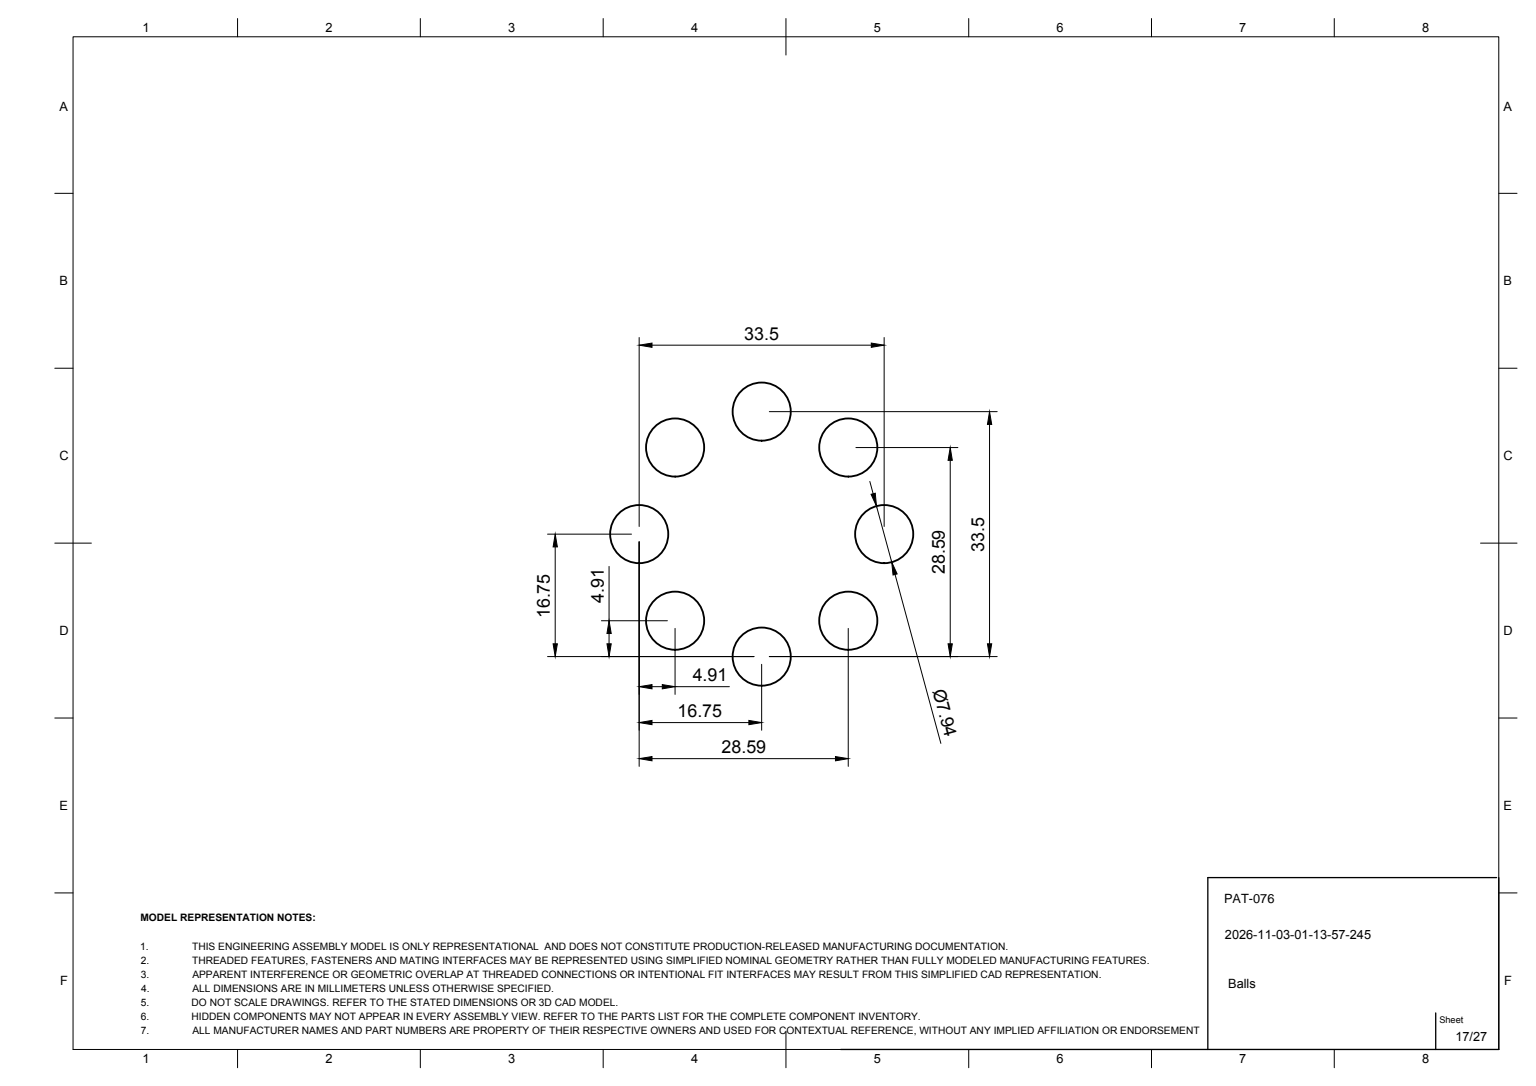
ISO-10303-21;
HEADER;
/* Generated by software containing ST-Developer
 * from STEP Tools, Inc. (www.steptools.com) 
 */

FILE_DESCRIPTION(
/* description */ ('Overhung pulley bearing cartridge'),
/* implementation_level */ '2;1');

FILE_NAME(
/* name */ 'Balls.step',
/* time_stamp */ '2026-10-28T03:22:33-07:00',
/* author */ (''),
/* organization */ (''),
/* preprocessor_version */ 'ST-DEVELOPER v20.2',
/* originating_system */ 'Autodesk Translation Framework v15.17.0.0',
/* authorisation */ '');

FILE_SCHEMA (('AUTOMOTIVE_DESIGN { 1 0 10303 214 3 1 1 }'));
ENDSEC;

DATA;
#10=MECHANICAL_DESIGN_GEOMETRIC_PRESENTATION_REPRESENTATION('',(#293,#294,#295,#296,#297,#298,#299,#300),#10963);
#207=SPHERICAL_SURFACE('',#6153,0.3969);
#208=SPHERICAL_SURFACE('',#6155,0.3969);
#209=SPHERICAL_SURFACE('',#6157,0.3969);
#210=SPHERICAL_SURFACE('',#6159,0.3969);
#211=SPHERICAL_SURFACE('',#6161,0.3969);
#212=SPHERICAL_SURFACE('',#6163,0.3969);
#213=SPHERICAL_SURFACE('',#6165,0.3969);
#214=SPHERICAL_SURFACE('',#6167,0.3969);
#249=SHAPE_REPRESENTATION_RELATIONSHIP('SRR','None',#11070,#271);
#271=ADVANCED_BREP_SHAPE_REPRESENTATION('',(#323,#324,#325,#326,#327,#328,
#329,#330),#10950);
#293=STYLED_ITEM('',(#11253),#323);
#294=STYLED_ITEM('',(#11253),#324);
#295=STYLED_ITEM('',(#11253),#325);
#296=STYLED_ITEM('',(#11253),#326);
#297=STYLED_ITEM('',(#11253),#327);
#298=STYLED_ITEM('',(#11253),#328);
#299=STYLED_ITEM('',(#11253),#329);
#300=STYLED_ITEM('',(#11253),#330);
#323=MANIFOLD_SOLID_BREP('Body1',#5660);
#324=MANIFOLD_SOLID_BREP('Body2',#5661);
#325=MANIFOLD_SOLID_BREP('Body3',#5662);
#326=MANIFOLD_SOLID_BREP('Body4',#5663);
#327=MANIFOLD_SOLID_BREP('Body5',#5664);
#328=MANIFOLD_SOLID_BREP('Body6',#5665);
#329=MANIFOLD_SOLID_BREP('Body7',#5666);
#330=MANIFOLD_SOLID_BREP('Body8',#5667);
#687=FACE_OUTER_BOUND('',#1075,.T.);
#688=FACE_OUTER_BOUND('',#1076,.T.);
#689=FACE_OUTER_BOUND('',#1077,.T.);
#690=FACE_OUTER_BOUND('',#1078,.T.);
#691=FACE_OUTER_BOUND('',#1079,.T.);
#692=FACE_OUTER_BOUND('',#1080,.T.);
#693=FACE_OUTER_BOUND('',#1081,.T.);
#694=FACE_OUTER_BOUND('',#1082,.T.);
#1075=EDGE_LOOP('',(#4099,#4100));
#1076=EDGE_LOOP('',(#4101,#4102));
#1077=EDGE_LOOP('',(#4103,#4104));
#1078=EDGE_LOOP('',(#4105,#4106));
#1079=EDGE_LOOP('',(#4107,#4108));
#1080=EDGE_LOOP('',(#4109,#4110));
#1081=EDGE_LOOP('',(#4111,#4112));
#1082=EDGE_LOOP('',(#4113,#4114));
#2116=CIRCLE('',#6154,0.3969);
#2117=CIRCLE('',#6156,0.3969);
#2118=CIRCLE('',#6158,0.3969);
#2119=CIRCLE('',#6160,0.3969);
#2120=CIRCLE('',#6162,0.3969);
#2121=CIRCLE('',#6164,0.3969);
#2122=CIRCLE('',#6166,0.3969);
#2123=CIRCLE('',#6168,0.3969);
#2529=VERTEX_POINT('',#9050);
#2530=VERTEX_POINT('',#9051);
#2531=VERTEX_POINT('',#9054);
#2532=VERTEX_POINT('',#9055);
#2533=VERTEX_POINT('',#9058);
#2534=VERTEX_POINT('',#9059);
#2535=VERTEX_POINT('',#9062);
#2536=VERTEX_POINT('',#9063);
#2537=VERTEX_POINT('',#9066);
#2538=VERTEX_POINT('',#9067);
#2539=VERTEX_POINT('',#9070);
#2540=VERTEX_POINT('',#9071);
#2541=VERTEX_POINT('',#9074);
#2542=VERTEX_POINT('',#9075);
#2543=VERTEX_POINT('',#9078);
#2544=VERTEX_POINT('',#9079);
#3119=EDGE_CURVE('',#2529,#2530,#2116,.T.);
#3120=EDGE_CURVE('',#2531,#2532,#2117,.T.);
#3121=EDGE_CURVE('',#2533,#2534,#2118,.T.);
#3122=EDGE_CURVE('',#2535,#2536,#2119,.T.);
#3123=EDGE_CURVE('',#2537,#2538,#2120,.T.);
#3124=EDGE_CURVE('',#2539,#2540,#2121,.T.);
#3125=EDGE_CURVE('',#2541,#2542,#2122,.T.);
#3126=EDGE_CURVE('',#2543,#2544,#2123,.T.);
#4099=ORIENTED_EDGE('',*,*,#3119,.T.);
#4100=ORIENTED_EDGE('',*,*,#3119,.F.);
#4101=ORIENTED_EDGE('',*,*,#3120,.T.);
#4102=ORIENTED_EDGE('',*,*,#3120,.F.);
#4103=ORIENTED_EDGE('',*,*,#3121,.T.);
#4104=ORIENTED_EDGE('',*,*,#3121,.F.);
#4105=ORIENTED_EDGE('',*,*,#3122,.T.);
#4106=ORIENTED_EDGE('',*,*,#3122,.F.);
#4107=ORIENTED_EDGE('',*,*,#3123,.T.);
#4108=ORIENTED_EDGE('',*,*,#3123,.F.);
#4109=ORIENTED_EDGE('',*,*,#3124,.T.);
#4110=ORIENTED_EDGE('',*,*,#3124,.F.);
#4111=ORIENTED_EDGE('',*,*,#3125,.T.);
#4112=ORIENTED_EDGE('',*,*,#3125,.F.);
#4113=ORIENTED_EDGE('',*,*,#3126,.T.);
#4114=ORIENTED_EDGE('',*,*,#3126,.F.);
#5431=ADVANCED_FACE('',(#687),#207,.T.);
#5432=ADVANCED_FACE('',(#688),#208,.T.);
#5433=ADVANCED_FACE('',(#689),#209,.T.);
#5434=ADVANCED_FACE('',(#690),#210,.T.);
#5435=ADVANCED_FACE('',(#691),#211,.T.);
#5436=ADVANCED_FACE('',(#692),#212,.T.);
#5437=ADVANCED_FACE('',(#693),#213,.T.);
#5438=ADVANCED_FACE('',(#694),#214,.T.);
#5660=CLOSED_SHELL('',(#5431));
#5661=CLOSED_SHELL('',(#5432));
#5662=CLOSED_SHELL('',(#5433));
#5663=CLOSED_SHELL('',(#5434));
#5664=CLOSED_SHELL('',(#5435));
#5665=CLOSED_SHELL('',(#5436));
#5666=CLOSED_SHELL('',(#5437));
#5667=CLOSED_SHELL('',(#5438));
#6152=AXIS2_PLACEMENT_3D('',#9048,#7261,#7262);
#6153=AXIS2_PLACEMENT_3D('',#9049,#7263,#7264);
#6154=AXIS2_PLACEMENT_3D('',#9052,#7265,#7266);
#6155=AXIS2_PLACEMENT_3D('',#9053,#7267,#7268);
#6156=AXIS2_PLACEMENT_3D('',#9056,#7269,#7270);
#6157=AXIS2_PLACEMENT_3D('',#9057,#7271,#7272);
#6158=AXIS2_PLACEMENT_3D('',#9060,#7273,#7274);
#6159=AXIS2_PLACEMENT_3D('',#9061,#7275,#7276);
#6160=AXIS2_PLACEMENT_3D('',#9064,#7277,#7278);
#6161=AXIS2_PLACEMENT_3D('',#9065,#7279,#7280);
#6162=AXIS2_PLACEMENT_3D('',#9068,#7281,#7282);
#6163=AXIS2_PLACEMENT_3D('',#9069,#7283,#7284);
#6164=AXIS2_PLACEMENT_3D('',#9072,#7285,#7286);
#6165=AXIS2_PLACEMENT_3D('',#9073,#7287,#7288);
#6166=AXIS2_PLACEMENT_3D('',#9076,#7289,#7290);
#6167=AXIS2_PLACEMENT_3D('',#9077,#7291,#7292);
#6168=AXIS2_PLACEMENT_3D('',#9080,#7293,#7294);
#7261=DIRECTION('axis',(0.,0.,1.));
#7262=DIRECTION('refdir',(1.,0.,0.));
#7263=DIRECTION('center_axis',(0.,0.,1.));
#7264=DIRECTION('ref_axis',(1.,0.,0.));
#7265=DIRECTION('center_axis',(1.22464679914735E-16,-1.,0.));
#7266=DIRECTION('ref_axis',(-1.,-1.22464679914735E-16,0.));
#7267=DIRECTION('center_axis',(0.707106781186548,0.,0.707106781186548));
#7268=DIRECTION('ref_axis',(0.707106781186548,0.,-0.707106781186548));
#7269=DIRECTION('center_axis',(8.65956056235493E-17,-1.,-8.65956056235493E-17));
#7270=DIRECTION('ref_axis',(-0.707106781186548,-1.22464679914735E-16,0.707106781186548));
#7271=DIRECTION('center_axis',(1.,0.,0.));
#7272=DIRECTION('ref_axis',(6.12323399573677E-17,0.,-1.));
#7273=DIRECTION('center_axis',(7.49879891330929E-33,-1.,-1.22464679914735E-16));
#7274=DIRECTION('ref_axis',(-6.12323399573677E-17,-1.22464679914735E-16,
1.));
#7275=DIRECTION('center_axis',(0.707106781186548,0.,-0.707106781186548));
#7276=DIRECTION('ref_axis',(-0.707106781186548,0.,-0.707106781186548));
#7277=DIRECTION('center_axis',(-8.65956056235493E-17,-1.,-8.65956056235493E-17));
#7278=DIRECTION('ref_axis',(0.707106781186548,-1.22464679914735E-16,0.707106781186548));
#7279=DIRECTION('center_axis',(0.,0.,-1.));
#7280=DIRECTION('ref_axis',(-1.,0.,-1.22464679914735E-16));
#7281=DIRECTION('center_axis',(-1.22464679914735E-16,-1.,-1.49975978266186E-32));
#7282=DIRECTION('ref_axis',(1.,-1.22464679914735E-16,1.22464679914735E-16));
#7283=DIRECTION('center_axis',(-0.707106781186548,0.,-0.707106781186548));
#7284=DIRECTION('ref_axis',(-0.707106781186548,0.,0.707106781186548));
#7285=DIRECTION('center_axis',(-8.65956056235493E-17,-1.,8.65956056235493E-17));
#7286=DIRECTION('ref_axis',(0.707106781186548,-1.22464679914735E-16,-0.707106781186548));
#7287=DIRECTION('center_axis',(-1.,0.,0.));
#7288=DIRECTION('ref_axis',(-1.83697019872103E-16,0.,1.));
#7289=DIRECTION('center_axis',(-2.24963967399279E-32,-1.,1.22464679914735E-16));
#7290=DIRECTION('ref_axis',(1.83697019872103E-16,-1.22464679914735E-16,
-1.));
#7291=DIRECTION('center_axis',(-0.707106781186548,0.,0.707106781186548));
#7292=DIRECTION('ref_axis',(0.707106781186548,0.,0.707106781186548));
#7293=DIRECTION('center_axis',(8.65956056235493E-17,-1.,8.65956056235494E-17));
#7294=DIRECTION('ref_axis',(-0.707106781186548,-1.22464679914735E-16,-0.707106781186548));
#9048=CARTESIAN_POINT('',(0.,0.,0.));
#9049=CARTESIAN_POINT('Origin',(1.675,0.,0.));
#9050=CARTESIAN_POINT('',(1.675,-2.97627328869245E-33,0.3969));
#9051=CARTESIAN_POINT('',(1.675,-2.97627328869245E-33,-0.3969));
#9052=CARTESIAN_POINT('Origin',(1.675,0.,0.));
#9053=CARTESIAN_POINT('Origin',(1.18440385848747,0.,-1.18440385848747));
#9054=CARTESIAN_POINT('',(1.46505453994041,3.1867025333467E-33,-0.903753177034526));
#9055=CARTESIAN_POINT('',(0.903753177034527,-9.13924911073161E-33,-1.46505453994041));
#9056=CARTESIAN_POINT('Origin',(1.18440385848747,0.,-1.18440385848747));
#9057=CARTESIAN_POINT('Origin',(1.02564169428591E-16,0.,-1.675));
#9058=CARTESIAN_POINT('',(0.3969,-2.97627328869246E-33,-1.675));
#9059=CARTESIAN_POINT('',(-0.3969,-2.97627328869245E-33,-1.675));
#9060=CARTESIAN_POINT('Origin',(1.02564169428591E-16,0.,-1.675));
#9061=CARTESIAN_POINT('Origin',(-1.18440385848747,0.,-1.18440385848747));
#9062=CARTESIAN_POINT('',(-0.903753177034526,3.1867025333467E-33,-1.46505453994041));
#9063=CARTESIAN_POINT('',(-1.46505453994041,-9.13924911073161E-33,-0.903753177034527));
#9064=CARTESIAN_POINT('Origin',(-1.18440385848747,0.,-1.18440385848747));
#9065=CARTESIAN_POINT('Origin',(-1.675,0.,-2.05128338857182E-16));
#9066=CARTESIAN_POINT('',(-1.675,-2.97627328869246E-33,-0.3969));
#9067=CARTESIAN_POINT('',(-1.675,-2.97627328869245E-33,0.3969));
#9068=CARTESIAN_POINT('Origin',(-1.675,0.,-2.05128338857182E-16));
#9069=CARTESIAN_POINT('Origin',(-1.18440385848747,0.,1.18440385848747));
#9070=CARTESIAN_POINT('',(-1.46505453994041,6.26819044436628E-33,0.903753177034526));
#9071=CARTESIAN_POINT('',(-0.903753177034527,-1.22207370217512E-32,1.46505453994041));
#9072=CARTESIAN_POINT('Origin',(-1.18440385848747,0.,1.18440385848747));
#9073=CARTESIAN_POINT('Origin',(-3.07692508285772E-16,0.,1.675));
#9074=CARTESIAN_POINT('',(-0.3969,-2.97627328869246E-33,1.675));
#9075=CARTESIAN_POINT('',(0.396899999999999,-2.97627328869245E-33,1.675));
#9076=CARTESIAN_POINT('Origin',(-3.07692508285772E-16,0.,1.675));
#9077=CARTESIAN_POINT('Origin',(1.18440385848747,0.,1.18440385848747));
#9078=CARTESIAN_POINT('',(0.903753177034526,9.34967835538585E-33,1.46505453994041));
#9079=CARTESIAN_POINT('',(1.46505453994041,-1.53022249327708E-32,0.903753177034527));
#9080=CARTESIAN_POINT('Origin',(1.18440385848747,0.,1.18440385848747));
#10923=UNCERTAINTY_MEASURE_WITH_UNIT(LENGTH_MEASURE(0.001),#10964,
'DISTANCE_ACCURACY_VALUE',
'Maximum model space distance between geometric entities at asserted c
onnectivities');
#10936=UNCERTAINTY_MEASURE_WITH_UNIT(LENGTH_MEASURE(0.001),#10964,
'DISTANCE_ACCURACY_VALUE',
'Maximum model space distance between geometric entities at asserted c
onnectivities');
#10950=(
GEOMETRIC_REPRESENTATION_CONTEXT(3)
GLOBAL_UNCERTAINTY_ASSIGNED_CONTEXT((#10923))
GLOBAL_UNIT_ASSIGNED_CONTEXT((#10964,#10966,#10967))
REPRESENTATION_CONTEXT('','3D')
);
#10963=(
GEOMETRIC_REPRESENTATION_CONTEXT(3)
GLOBAL_UNCERTAINTY_ASSIGNED_CONTEXT((#10936))
GLOBAL_UNIT_ASSIGNED_CONTEXT((#10964,#10966,#10967))
REPRESENTATION_CONTEXT('','3D')
);
#10964=(
LENGTH_UNIT()
NAMED_UNIT(*)
SI_UNIT(.CENTI.,.METRE.)
);
#10966=(
NAMED_UNIT(*)
PLANE_ANGLE_UNIT()
SI_UNIT($,.RADIAN.)
);
#10967=(
NAMED_UNIT(*)
SI_UNIT($,.STERADIAN.)
SOLID_ANGLE_UNIT()
);
#10981=SHAPE_DEFINITION_REPRESENTATION(#11007,#11070);
#11007=PRODUCT_DEFINITION_SHAPE('',$,#11097);
#11070=SHAPE_REPRESENTATION('',(#6152),#10950);
#11083=PRODUCT_DEFINITION_CONTEXT('part definition',#11163,'design');
#11097=PRODUCT_DEFINITION('Balls','Balls',#11123,#11083);
#11123=PRODUCT_DEFINITION_FORMATION('',$,#11178);
#11163=APPLICATION_CONTEXT(
'Core Data for Automotive Mechanical Design Process');
#11164=PRODUCT_CONTEXT('part definition',#11163,'mechanical');
#11178=PRODUCT('Balls','Balls','Balls',(#11164));
#11247=COLOUR_RGB('Grey',0.48,0.52,0.57);
#11248=FILL_AREA_STYLE_COLOUR('',#11247);
#11249=FILL_AREA_STYLE('',(#11248));
#11250=SURFACE_STYLE_FILL_AREA(#11249);
#11251=SURFACE_SIDE_STYLE('',(#11250));
#11252=SURFACE_STYLE_USAGE(.BOTH.,#11251);
#11253=PRESENTATION_STYLE_ASSIGNMENT((#11252));
ENDSEC;
END-ISO-10303-21;
